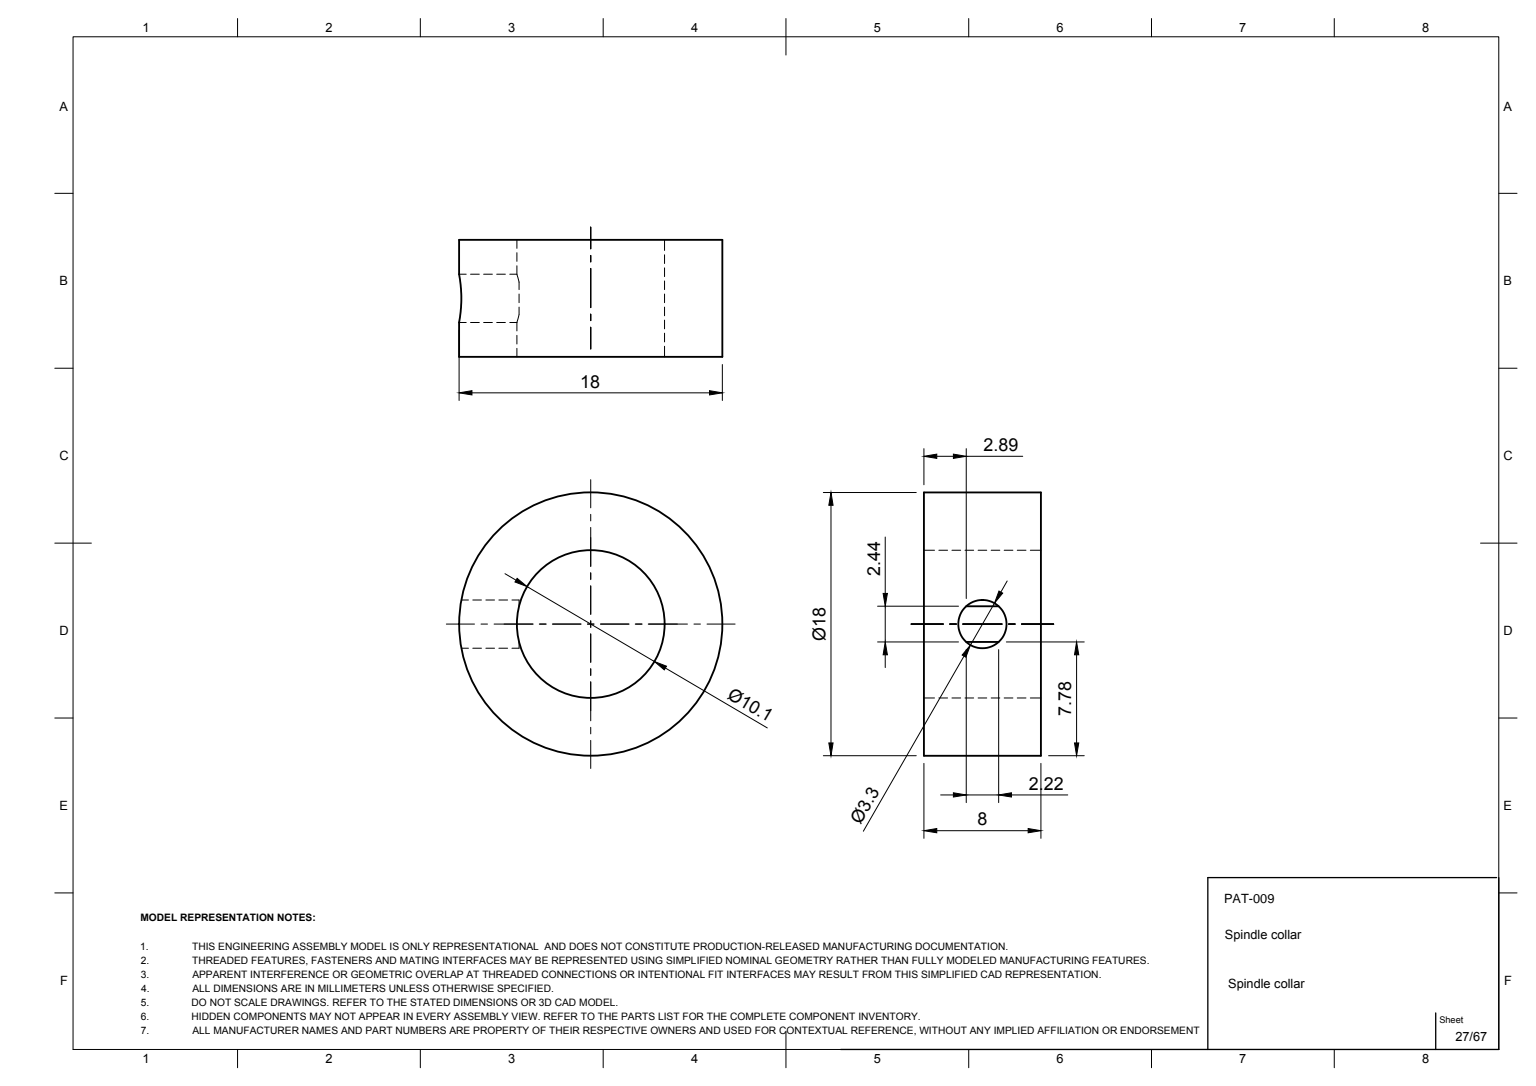
ISO-10303-21;
HEADER;
/* Generated by software containing ST-Developer
 * from STEP Tools, Inc. (www.steptools.com) 
 */

FILE_DESCRIPTION(
/* description */ ('Bell-crank linkage with push rods'),
/* implementation_level */ '2;1');

FILE_NAME(
/* name */ 'Spindle collar.step',
/* time_stamp */ '2026-10-28T03:25:15-07:00',
/* author */ (''),
/* organization */ (''),
/* preprocessor_version */ 'ST-DEVELOPER v20.2',
/* originating_system */ 'Autodesk Translation Framework v15.17.0.0',
/* authorisation */ '');

FILE_SCHEMA (('AUTOMOTIVE_DESIGN { 1 0 10303 214 3 1 1 }'));
ENDSEC;

DATA;
#10=MECHANICAL_DESIGN_GEOMETRIC_PRESENTATION_REPRESENTATION('',(#632),#16678);
#491=B_SPLINE_CURVE_WITH_KNOTS('',3,(#15275,#15276,#15277,#15278,#15279,
#15280,#15281,#15282,#15283,#15284,#15285,#15286,#15287,#15288),
 .UNSPECIFIED.,.F.,.F.,(4,2,2,2,2,2,4),(0.618551524396293,0.626563103102765,
0.689203386094988,0.751843669087211,0.814483952079434,0.877124235071657,
0.88513581377813),.UNSPECIFIED.);
#492=B_SPLINE_CURVE_WITH_KNOTS('',3,(#15292,#15293,#15294,#15295,#15296,
#15297,#15298,#15299),.UNSPECIFIED.,.F.,.F.,(4,2,2,4),(0.250614556362404,
0.313254839354627,0.37589512234685,0.383906701053323),.UNSPECIFIED.);
#493=B_SPLINE_CURVE_WITH_KNOTS('',3,(#15303,#15304,#15305,#15306,#15307,
#15308,#15309,#15310,#15311,#15312,#15313,#15314,#15315,#15316,#15317,#15318,
#15319,#15320,#15321,#15322,#15323,#15324,#15325,#15326,#15327,#15328),
 .UNSPECIFIED.,.F.,.F.,(4,2,2,2,2,2,2,2,2,2,2,2,4),(0.,0.0623062782223143,
0.124612556444629,0.186916384615149,0.249220212785669,0.31152404095619,
0.37382786912671,0.436134147349024,0.498440425571339,0.560746703793653,
0.623052982015967,0.685356810186488,0.747660638357008),.UNSPECIFIED.);
#494=B_SPLINE_CURVE_WITH_KNOTS('',3,(#15329,#15330,#15331,#15332,#15333,
#15334,#15335,#15336,#15337,#15338),.UNSPECIFIED.,.F.,.F.,(4,2,2,2,4),(0.747660638357008,
0.809964466527528,0.872268294698049,0.934574572920363,0.996880851142677),
 .UNSPECIFIED.);
#495=B_SPLINE_CURVE_WITH_KNOTS('',3,(#15339,#15340,#15341,#15342,#15343,
#15344,#15345,#15346),.UNSPECIFIED.,.F.,.F.,(4,2,2,4),(0.117322411671485,
0.125333990377958,0.187974273370181,0.250614556362404),.UNSPECIFIED.);
#516=SHAPE_REPRESENTATION_RELATIONSHIP('SRR','None',#16934,#570);
#570=ADVANCED_BREP_SHAPE_REPRESENTATION('',(#693),#16639);
#632=STYLED_ITEM('',(#17284),#693);
#693=MANIFOLD_SOLID_BREP('Body1',#8823);
#834=FACE_BOUND('',#2142,.T.);
#835=FACE_BOUND('',#2144,.T.);
#836=FACE_BOUND('',#2146,.T.);
#837=FACE_BOUND('',#2148,.T.);
#1097=PLANE('',#10012);
#1098=PLANE('',#10016);
#1099=PLANE('',#10023);
#1100=PLANE('',#10024);
#1507=FACE_OUTER_BOUND('',#2138,.T.);
#1508=FACE_OUTER_BOUND('',#2139,.T.);
#1509=FACE_OUTER_BOUND('',#2140,.T.);
#1510=FACE_OUTER_BOUND('',#2141,.T.);
#1511=FACE_OUTER_BOUND('',#2143,.T.);
#1512=FACE_OUTER_BOUND('',#2145,.T.);
#1513=FACE_OUTER_BOUND('',#2147,.T.);
#2138=EDGE_LOOP('',(#7073,#7074));
#2139=EDGE_LOOP('',(#7075,#7076,#7077,#7078,#7079,#7080,#7081,#7082,#7083));
#2140=EDGE_LOOP('',(#7084,#7085));
#2141=EDGE_LOOP('',(#7086,#7087,#7088,#7089));
#2142=EDGE_LOOP('',(#7090,#7091,#7092,#7093,#7094));
#2143=EDGE_LOOP('',(#7095,#7096,#7097,#7098));
#2144=EDGE_LOOP('',(#7099,#7100));
#2145=EDGE_LOOP('',(#7101));
#2146=EDGE_LOOP('',(#7102));
#2147=EDGE_LOOP('',(#7103));
#2148=EDGE_LOOP('',(#7104));
#2811=LINE('',#15271,#3360);
#2812=LINE('',#15301,#3361);
#2813=LINE('',#15348,#3362);
#2814=LINE('',#15353,#3363);
#2815=LINE('',#15359,#3364);
#3360=VECTOR('',#12027,1.);
#3361=VECTOR('',#12034,0.165);
#3362=VECTOR('',#12037,1.);
#3363=VECTOR('',#12042,0.505);
#3364=VECTOR('',#12049,0.9);
#3898=CIRCLE('',#10013,0.165);
#3899=CIRCLE('',#10015,0.165);
#3900=CIRCLE('',#10018,0.505);
#3901=CIRCLE('',#10019,0.505);
#3902=CIRCLE('',#10021,0.9);
#3903=CIRCLE('',#10022,0.9);
#4504=VERTEX_POINT('',#15269);
#4505=VERTEX_POINT('',#15270);
#4506=VERTEX_POINT('',#15274);
#4507=VERTEX_POINT('',#15289);
#4508=VERTEX_POINT('',#15291);
#4509=VERTEX_POINT('',#15300);
#4510=VERTEX_POINT('',#15302);
#4511=VERTEX_POINT('',#15350);
#4512=VERTEX_POINT('',#15352);
#4513=VERTEX_POINT('',#15356);
#4514=VERTEX_POINT('',#15358);
#5414=EDGE_CURVE('',#4504,#4505,#2811,.T.);
#5415=EDGE_CURVE('',#4504,#4505,#3898,.T.);
#5416=EDGE_CURVE('',#4506,#4504,#491,.T.);
#5417=EDGE_CURVE('',#4507,#4506,#3899,.T.);
#5418=EDGE_CURVE('',#4508,#4507,#492,.T.);
#5419=EDGE_CURVE('',#4508,#4509,#2812,.T.);
#5420=EDGE_CURVE('',#4510,#4509,#493,.T.);
#5421=EDGE_CURVE('',#4509,#4510,#494,.T.);
#5422=EDGE_CURVE('',#4505,#4508,#495,.T.);
#5423=EDGE_CURVE('',#4507,#4506,#2813,.T.);
#5424=EDGE_CURVE('',#4511,#4511,#3900,.T.);
#5425=EDGE_CURVE('',#4511,#4512,#2814,.T.);
#5426=EDGE_CURVE('',#4512,#4512,#3901,.T.);
#5427=EDGE_CURVE('',#4513,#4513,#3902,.T.);
#5428=EDGE_CURVE('',#4513,#4514,#2815,.T.);
#5429=EDGE_CURVE('',#4514,#4514,#3903,.T.);
#7073=ORIENTED_EDGE('',*,*,#5414,.F.);
#7074=ORIENTED_EDGE('',*,*,#5415,.T.);
#7075=ORIENTED_EDGE('',*,*,#5416,.F.);
#7076=ORIENTED_EDGE('',*,*,#5417,.F.);
#7077=ORIENTED_EDGE('',*,*,#5418,.F.);
#7078=ORIENTED_EDGE('',*,*,#5419,.T.);
#7079=ORIENTED_EDGE('',*,*,#5420,.F.);
#7080=ORIENTED_EDGE('',*,*,#5421,.F.);
#7081=ORIENTED_EDGE('',*,*,#5419,.F.);
#7082=ORIENTED_EDGE('',*,*,#5422,.F.);
#7083=ORIENTED_EDGE('',*,*,#5415,.F.);
#7084=ORIENTED_EDGE('',*,*,#5423,.F.);
#7085=ORIENTED_EDGE('',*,*,#5417,.T.);
#7086=ORIENTED_EDGE('',*,*,#5424,.F.);
#7087=ORIENTED_EDGE('',*,*,#5425,.T.);
#7088=ORIENTED_EDGE('',*,*,#5426,.T.);
#7089=ORIENTED_EDGE('',*,*,#5425,.F.);
#7090=ORIENTED_EDGE('',*,*,#5422,.T.);
#7091=ORIENTED_EDGE('',*,*,#5418,.T.);
#7092=ORIENTED_EDGE('',*,*,#5423,.T.);
#7093=ORIENTED_EDGE('',*,*,#5416,.T.);
#7094=ORIENTED_EDGE('',*,*,#5414,.T.);
#7095=ORIENTED_EDGE('',*,*,#5427,.F.);
#7096=ORIENTED_EDGE('',*,*,#5428,.T.);
#7097=ORIENTED_EDGE('',*,*,#5429,.T.);
#7098=ORIENTED_EDGE('',*,*,#5428,.F.);
#7099=ORIENTED_EDGE('',*,*,#5420,.T.);
#7100=ORIENTED_EDGE('',*,*,#5421,.T.);
#7101=ORIENTED_EDGE('',*,*,#5427,.T.);
#7102=ORIENTED_EDGE('',*,*,#5424,.T.);
#7103=ORIENTED_EDGE('',*,*,#5429,.F.);
#7104=ORIENTED_EDGE('',*,*,#5426,.F.);
#8168=CYLINDRICAL_SURFACE('',#10014,0.165);
#8169=CYLINDRICAL_SURFACE('',#10017,0.505);
#8170=CYLINDRICAL_SURFACE('',#10020,0.9);
#8532=ADVANCED_FACE('',(#1507),#1097,.T.);
#8533=ADVANCED_FACE('',(#1508),#8168,.F.);
#8534=ADVANCED_FACE('',(#1509),#1098,.T.);
#8535=ADVANCED_FACE('',(#1510,#834),#8169,.F.);
#8536=ADVANCED_FACE('',(#1511,#835),#8170,.T.);
#8537=ADVANCED_FACE('',(#1512,#836),#1099,.T.);
#8538=ADVANCED_FACE('',(#1513,#837),#1100,.F.);
#8823=CLOSED_SHELL('',(#8532,#8533,#8534,#8535,#8536,#8537,#8538));
#10011=AXIS2_PLACEMENT_3D('',#15267,#12023,#12024);
#10012=AXIS2_PLACEMENT_3D('',#15268,#12025,#12026);
#10013=AXIS2_PLACEMENT_3D('',#15272,#12028,#12029);
#10014=AXIS2_PLACEMENT_3D('',#15273,#12030,#12031);
#10015=AXIS2_PLACEMENT_3D('',#15290,#12032,#12033);
#10016=AXIS2_PLACEMENT_3D('',#15347,#12035,#12036);
#10017=AXIS2_PLACEMENT_3D('',#15349,#12038,#12039);
#10018=AXIS2_PLACEMENT_3D('',#15351,#12040,#12041);
#10019=AXIS2_PLACEMENT_3D('',#15354,#12043,#12044);
#10020=AXIS2_PLACEMENT_3D('',#15355,#12045,#12046);
#10021=AXIS2_PLACEMENT_3D('',#15357,#12047,#12048);
#10022=AXIS2_PLACEMENT_3D('',#15360,#12050,#12051);
#10023=AXIS2_PLACEMENT_3D('',#15361,#12052,#12053);
#10024=AXIS2_PLACEMENT_3D('',#15362,#12054,#12055);
#12023=DIRECTION('axis',(0.,0.,1.));
#12024=DIRECTION('refdir',(1.,0.,0.));
#12025=DIRECTION('center_axis',(1.,0.,0.));
#12026=DIRECTION('ref_axis',(0.,0.,-1.));
#12027=DIRECTION('',(0.,0.,1.));
#12028=DIRECTION('center_axis',(1.,0.,0.));
#12029=DIRECTION('ref_axis',(0.,0.,-1.));
#12030=DIRECTION('center_axis',(1.,0.,0.));
#12031=DIRECTION('ref_axis',(0.,0.,-1.));
#12032=DIRECTION('center_axis',(1.,0.,0.));
#12033=DIRECTION('ref_axis',(0.,0.,-1.));
#12034=DIRECTION('',(1.,0.,0.));
#12035=DIRECTION('center_axis',(1.,0.,0.));
#12036=DIRECTION('ref_axis',(0.,0.,-1.));
#12037=DIRECTION('',(0.,0.,-1.));
#12038=DIRECTION('center_axis',(0.,0.,1.));
#12039=DIRECTION('ref_axis',(1.,0.,0.));
#12040=DIRECTION('center_axis',(0.,0.,-1.));
#12041=DIRECTION('ref_axis',(1.,0.,0.));
#12042=DIRECTION('',(0.,0.,-1.));
#12043=DIRECTION('center_axis',(0.,0.,-1.));
#12044=DIRECTION('ref_axis',(1.,0.,0.));
#12045=DIRECTION('center_axis',(0.,0.,1.));
#12046=DIRECTION('ref_axis',(1.,0.,0.));
#12047=DIRECTION('center_axis',(0.,0.,1.));
#12048=DIRECTION('ref_axis',(1.,0.,0.));
#12049=DIRECTION('',(0.,0.,-1.));
#12050=DIRECTION('center_axis',(0.,0.,1.));
#12051=DIRECTION('ref_axis',(1.,0.,0.));
#12052=DIRECTION('center_axis',(0.,0.,1.));
#12053=DIRECTION('ref_axis',(1.,0.,0.));
#12054=DIRECTION('center_axis',(0.,0.,1.));
#12055=DIRECTION('ref_axis',(1.,0.,0.));
#15267=CARTESIAN_POINT('',(0.,0.,0.));
#15268=CARTESIAN_POINT('Origin',(0.49,0.,1.4));
#15269=CARTESIAN_POINT('',(0.49,0.122167917228706,1.28909463493591));
#15270=CARTESIAN_POINT('',(0.49,0.122167917228706,1.51090536506409));
#15271=CARTESIAN_POINT('',(0.49,0.122167917228706,1.));
#15272=CARTESIAN_POINT('Origin',(0.49,0.,1.4));
#15273=CARTESIAN_POINT('Origin',(0.49,0.,1.4));
#15274=CARTESIAN_POINT('',(0.49,-0.122167917228706,1.28909463493591));
#15275=CARTESIAN_POINT('Ctrl Pts',(0.49,-0.122167917228706,1.28909463493591));
#15276=CARTESIAN_POINT('Ctrl Pts',(0.490448531679987,-0.120368913626296,
1.28711294069536));
#15277=CARTESIAN_POINT('Ctrl Pts',(0.490895245371685,-0.118534896565231,
1.28518965877367));
#15278=CARTESIAN_POINT('Ctrl Pts',(0.494795015531646,-0.102111993019358,
1.2687667552278));
#15279=CARTESIAN_POINT('Ctrl Pts',(0.498442514607594,-0.0836597150224318,
1.25609154388858));
#15280=CARTESIAN_POINT('Ctrl Pts',(0.50357781976106,-0.0430495960471595,
1.23920409039234));
#15281=CARTESIAN_POINT('Ctrl Pts',(0.505,-0.020880094330741,1.235));
#15282=CARTESIAN_POINT('Ctrl Pts',(0.505,0.020880094330741,1.235));
#15283=CARTESIAN_POINT('Ctrl Pts',(0.50357781976106,0.0430495960471595,
1.23920409039234));
#15284=CARTESIAN_POINT('Ctrl Pts',(0.498442514607594,0.0836597150224318,
1.25609154388858));
#15285=CARTESIAN_POINT('Ctrl Pts',(0.494795015531646,0.102111993019358,
1.2687667552278));
#15286=CARTESIAN_POINT('Ctrl Pts',(0.490895245371684,0.118534896565231,
1.28518965877367));
#15287=CARTESIAN_POINT('Ctrl Pts',(0.490448531679987,0.120368913626296,
1.28711294069536));
#15288=CARTESIAN_POINT('Ctrl Pts',(0.49,0.122167917228706,1.28909463493591));
#15289=CARTESIAN_POINT('',(0.49,-0.122167917228706,1.51090536506409));
#15290=CARTESIAN_POINT('Origin',(0.49,0.,1.4));
#15291=CARTESIAN_POINT('',(0.505,-1.70422299968729E-17,1.565));
#15292=CARTESIAN_POINT('Ctrl Pts',(0.505,-6.93889390390723E-18,1.565));
#15293=CARTESIAN_POINT('Ctrl Pts',(0.505,-0.020880094330741,1.565));
#15294=CARTESIAN_POINT('Ctrl Pts',(0.50357781976106,-0.0430495960471595,
1.56079590960766));
#15295=CARTESIAN_POINT('Ctrl Pts',(0.498442514607594,-0.0836597150224318,
1.54390845611142));
#15296=CARTESIAN_POINT('Ctrl Pts',(0.494795015531646,-0.102111993019358,
1.5312332447722));
#15297=CARTESIAN_POINT('Ctrl Pts',(0.490895245371684,-0.118534896565231,
1.51481034122633));
#15298=CARTESIAN_POINT('Ctrl Pts',(0.490448531679987,-0.120368913626296,
1.51288705930464));
#15299=CARTESIAN_POINT('Ctrl Pts',(0.49,-0.122167917228706,1.51090536506409));
#15300=CARTESIAN_POINT('',(0.9,-2.02066721859313E-17,1.565));
#15301=CARTESIAN_POINT('',(0.49,-2.02066721859313E-17,1.565));
#15302=CARTESIAN_POINT('',(0.884745726183518,0.165,1.4));
#15303=CARTESIAN_POINT('Ctrl Pts',(0.884745726183518,0.165,1.4));
#15304=CARTESIAN_POINT('Ctrl Pts',(0.884745726183518,0.165,1.37923124059256));
#15305=CARTESIAN_POINT('Ctrl Pts',(0.885552759505264,0.160839719007584,
1.35711110492666));
#15306=CARTESIAN_POINT('Ctrl Pts',(0.888448648150043,0.143986470216691,
1.31647293736623));
#15307=CARTESIAN_POINT('Ctrl Pts',(0.890493604851638,0.131295993814186,
1.29795075602263));
#15308=CARTESIAN_POINT('Ctrl Pts',(0.89431723432394,0.102049819008125,1.26870458121656));
#15309=CARTESIAN_POINT('Ctrl Pts',(0.896347088899543,0.0835273920906824,
1.25601365401642));
#15310=CARTESIAN_POINT('Ctrl Pts',(0.899208271860583,0.0428883760934127,
1.23916007816136));
#15311=CARTESIAN_POINT('Ctrl Pts',(0.9,0.0207679427235068,1.235));
#15312=CARTESIAN_POINT('Ctrl Pts',(0.9,-0.0207679427235068,1.235));
#15313=CARTESIAN_POINT('Ctrl Pts',(0.899208271860583,-0.0428883760934127,
1.23916007816136));
#15314=CARTESIAN_POINT('Ctrl Pts',(0.896347088899543,-0.0835273920906823,
1.25601365401642));
#15315=CARTESIAN_POINT('Ctrl Pts',(0.89431723432394,-0.102049819008125,
1.26870458121656));
#15316=CARTESIAN_POINT('Ctrl Pts',(0.890493604851638,-0.131295993814186,
1.29795075602263));
#15317=CARTESIAN_POINT('Ctrl Pts',(0.888448648150043,-0.143986470216691,
1.31647293736623));
#15318=CARTESIAN_POINT('Ctrl Pts',(0.885552759505264,-0.160839719007584,
1.35711110492666));
#15319=CARTESIAN_POINT('Ctrl Pts',(0.884745726183518,-0.165,1.37923124059256));
#15320=CARTESIAN_POINT('Ctrl Pts',(0.884745726183518,-0.165,1.42076875940744));
#15321=CARTESIAN_POINT('Ctrl Pts',(0.885552759505264,-0.160839719007584,
1.44288889507334));
#15322=CARTESIAN_POINT('Ctrl Pts',(0.888448648150043,-0.14398647021669,
1.48352706263377));
#15323=CARTESIAN_POINT('Ctrl Pts',(0.890493604851638,-0.131295993814186,
1.50204924397737));
#15324=CARTESIAN_POINT('Ctrl Pts',(0.89431723432394,-0.102049819008125,
1.53129541878344));
#15325=CARTESIAN_POINT('Ctrl Pts',(0.896347088899543,-0.0835273920906824,
1.54398634598358));
#15326=CARTESIAN_POINT('Ctrl Pts',(0.899208271860583,-0.0428883760934128,
1.56083992183864));
#15327=CARTESIAN_POINT('Ctrl Pts',(0.9,-0.0207679427235068,1.565));
#15328=CARTESIAN_POINT('Ctrl Pts',(0.9,-6.93889390390723E-18,1.565));
#15329=CARTESIAN_POINT('Ctrl Pts',(0.9,-3.46944695195361E-17,1.565));
#15330=CARTESIAN_POINT('Ctrl Pts',(0.9,0.0207679427235068,1.565));
#15331=CARTESIAN_POINT('Ctrl Pts',(0.899208271860583,0.0428883760934127,
1.56083992183864));
#15332=CARTESIAN_POINT('Ctrl Pts',(0.896347088899543,0.0835273920906824,
1.54398634598358));
#15333=CARTESIAN_POINT('Ctrl Pts',(0.89431723432394,0.102049819008125,1.53129541878344));
#15334=CARTESIAN_POINT('Ctrl Pts',(0.890493604851638,0.131295993814186,
1.50204924397737));
#15335=CARTESIAN_POINT('Ctrl Pts',(0.888448648150043,0.143986470216691,
1.48352706263377));
#15336=CARTESIAN_POINT('Ctrl Pts',(0.885552759505264,0.160839719007584,
1.44288889507334));
#15337=CARTESIAN_POINT('Ctrl Pts',(0.884745726183518,0.165,1.42076875940744));
#15338=CARTESIAN_POINT('Ctrl Pts',(0.884745726183518,0.165,1.4));
#15339=CARTESIAN_POINT('Ctrl Pts',(0.49,0.122167917228706,1.51090536506409));
#15340=CARTESIAN_POINT('Ctrl Pts',(0.490448531679987,0.120368913626296,
1.51288705930464));
#15341=CARTESIAN_POINT('Ctrl Pts',(0.490895245371685,0.118534896565231,
1.51481034122633));
#15342=CARTESIAN_POINT('Ctrl Pts',(0.494795015531646,0.102111993019358,
1.5312332447722));
#15343=CARTESIAN_POINT('Ctrl Pts',(0.498442514607594,0.0836597150224318,
1.54390845611142));
#15344=CARTESIAN_POINT('Ctrl Pts',(0.50357781976106,0.0430495960471594,
1.56079590960766));
#15345=CARTESIAN_POINT('Ctrl Pts',(0.505,0.020880094330741,1.565));
#15346=CARTESIAN_POINT('Ctrl Pts',(0.505,0.,1.565));
#15347=CARTESIAN_POINT('Origin',(0.49,0.,1.4));
#15348=CARTESIAN_POINT('',(0.49,-0.122167917228706,1.));
#15349=CARTESIAN_POINT('Origin',(0.,0.,1.));
#15350=CARTESIAN_POINT('',(-0.505,-6.18446633569413E-17,1.8));
#15351=CARTESIAN_POINT('Origin',(0.,0.,1.8));
#15352=CARTESIAN_POINT('',(-0.505,-6.18446633569413E-17,1.));
#15353=CARTESIAN_POINT('',(-0.505,-6.18446633569413E-17,1.));
#15354=CARTESIAN_POINT('Origin',(0.,0.,1.));
#15355=CARTESIAN_POINT('Origin',(0.,0.,1.));
#15356=CARTESIAN_POINT('',(-0.9,-1.10218211923262E-16,1.8));
#15357=CARTESIAN_POINT('Origin',(0.,0.,1.8));
#15358=CARTESIAN_POINT('',(-0.9,-1.10218211923262E-16,1.));
#15359=CARTESIAN_POINT('',(-0.9,-1.10218211923262E-16,1.));
#15360=CARTESIAN_POINT('Origin',(0.,0.,1.));
#15361=CARTESIAN_POINT('Origin',(0.,0.,1.8));
#15362=CARTESIAN_POINT('Origin',(0.,0.,1.));
#16575=UNCERTAINTY_MEASURE_WITH_UNIT(LENGTH_MEASURE(0.001),#16679,
'DISTANCE_ACCURACY_VALUE',
'Maximum model space distance between geometric entities at asserted c
onnectivities');
#16614=UNCERTAINTY_MEASURE_WITH_UNIT(LENGTH_MEASURE(0.001),#16679,
'DISTANCE_ACCURACY_VALUE',
'Maximum model space distance between geometric entities at asserted c
onnectivities');
#16639=(
GEOMETRIC_REPRESENTATION_CONTEXT(3)
GLOBAL_UNCERTAINTY_ASSIGNED_CONTEXT((#16575))
GLOBAL_UNIT_ASSIGNED_CONTEXT((#16679,#16681,#16682))
REPRESENTATION_CONTEXT('','3D')
);
#16678=(
GEOMETRIC_REPRESENTATION_CONTEXT(3)
GLOBAL_UNCERTAINTY_ASSIGNED_CONTEXT((#16614))
GLOBAL_UNIT_ASSIGNED_CONTEXT((#16679,#16681,#16682))
REPRESENTATION_CONTEXT('','3D')
);
#16679=(
LENGTH_UNIT()
NAMED_UNIT(*)
SI_UNIT(.CENTI.,.METRE.)
);
#16681=(
NAMED_UNIT(*)
PLANE_ANGLE_UNIT()
SI_UNIT($,.RADIAN.)
);
#16682=(
NAMED_UNIT(*)
SI_UNIT($,.STERADIAN.)
SOLID_ANGLE_UNIT()
);
#16707=SHAPE_DEFINITION_REPRESENTATION(#16775,#16934);
#16775=PRODUCT_DEFINITION_SHAPE('',$,#16998);
#16934=SHAPE_REPRESENTATION('',(#10011),#16639);
#16973=PRODUCT_DEFINITION_CONTEXT('part definition',#17164,'design');
#16998=PRODUCT_DEFINITION('Spindle collar','Spindle collar',#17061,#16973);
#17061=PRODUCT_DEFINITION_FORMATION('',$,#17190);
#17164=APPLICATION_CONTEXT(
'Core Data for Automotive Mechanical Design Process');
#17165=PRODUCT_CONTEXT('part definition',#17164,'mechanical');
#17190=PRODUCT('Spindle collar','Spindle collar','Spindle collar',(#17165));
#17278=COLOUR_RGB('Sky Blue',0.24,0.69,0.87);
#17279=FILL_AREA_STYLE_COLOUR('',#17278);
#17280=FILL_AREA_STYLE('',(#17279));
#17281=SURFACE_STYLE_FILL_AREA(#17280);
#17282=SURFACE_SIDE_STYLE('',(#17281));
#17283=SURFACE_STYLE_USAGE(.BOTH.,#17282);
#17284=PRESENTATION_STYLE_ASSIGNMENT((#17283));
ENDSEC;
END-ISO-10303-21;
